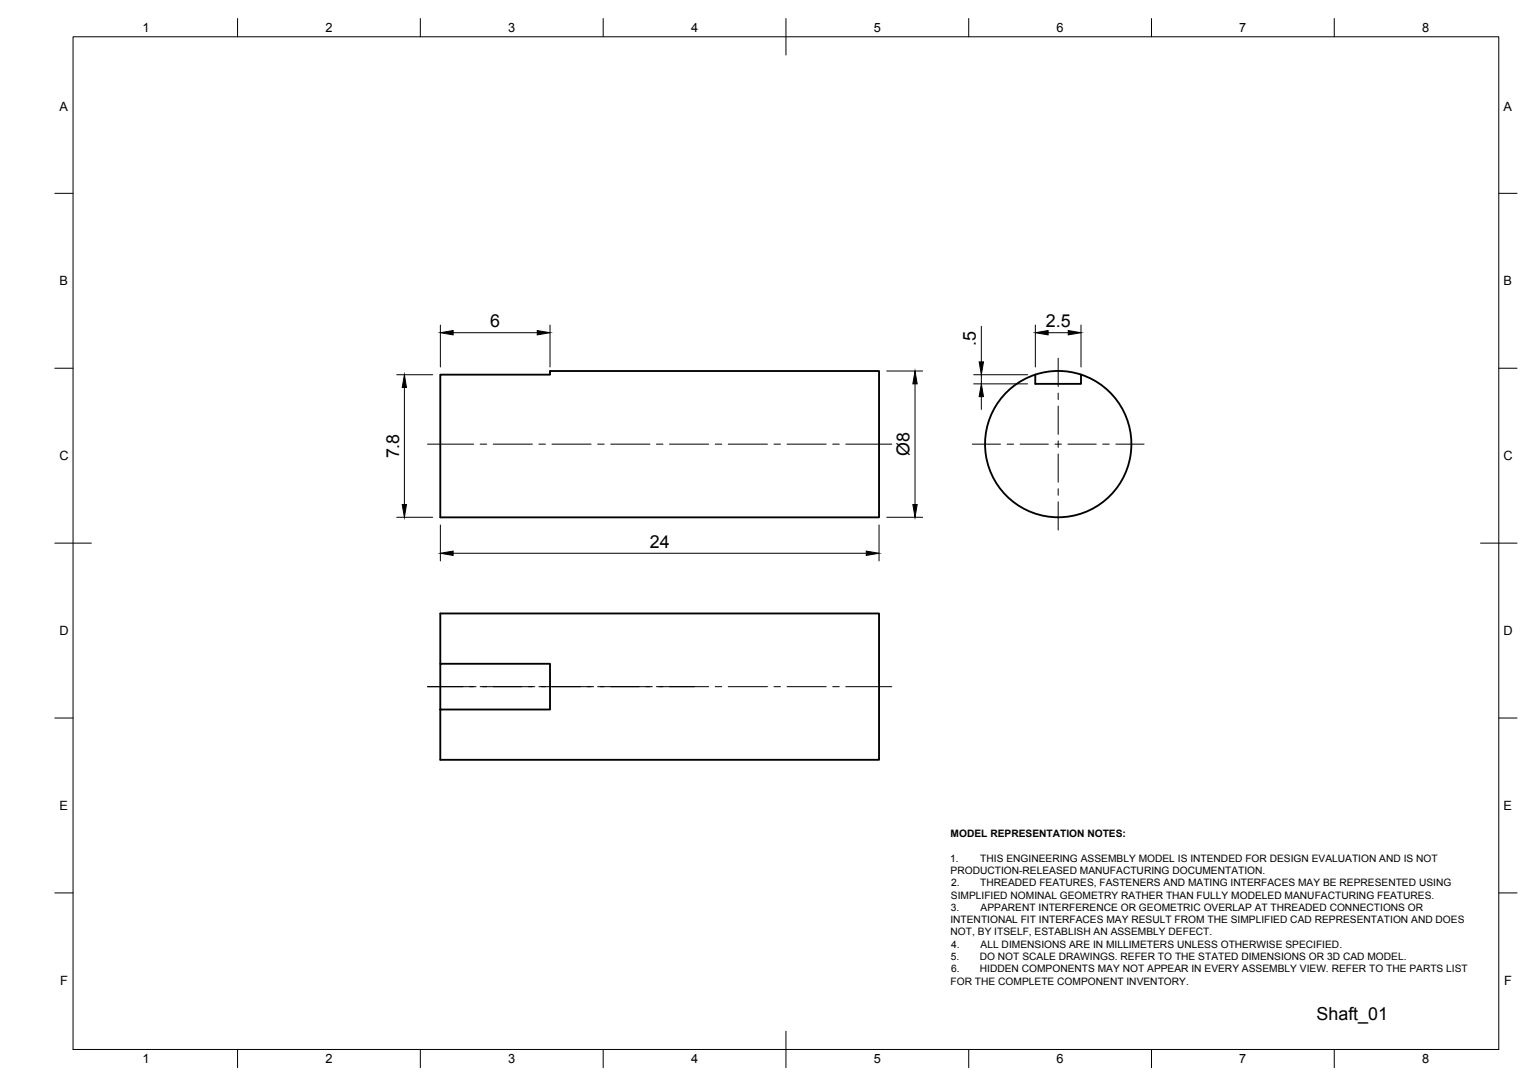
ISO-10303-21;
HEADER;
/* Generated by software containing ST-Developer
 * from STEP Tools, Inc. (www.steptools.com) 
 */

FILE_DESCRIPTION(
/* description */ (''),
/* implementation_level */ '2;1');

FILE_NAME(
/* name */ 'Shaft_01.step',
/* time_stamp */ '2026-10-05T22:24:12-07:00',
/* author */ (''),
/* organization */ (''),
/* preprocessor_version */ 'ST-DEVELOPER v20.2',
/* originating_system */ 'Autodesk Translation Framework v15.15.0.0',
/* authorisation */ '');

FILE_SCHEMA (('AUTOMOTIVE_DESIGN { 1 0 10303 214 3 1 1 }'));
ENDSEC;

DATA;
#10=MECHANICAL_DESIGN_GEOMETRIC_PRESENTATION_REPRESENTATION('',(#58),#2116);
#44=SHAPE_REPRESENTATION_RELATIONSHIP('SRR','None',#2150,#51);
#51=ADVANCED_BREP_SHAPE_REPRESENTATION('',(#65),#2114);
#58=STYLED_ITEM('',(#2192),#65);
#65=MANIFOLD_SOLID_BREP('Body1',#1152);
#119=PLANE('',#1329);
#120=PLANE('',#1330);
#121=PLANE('',#1332);
#122=PLANE('',#1333);
#123=PLANE('',#1338);
#124=PLANE('',#1339);
#185=FACE_OUTER_BOUND('',#260,.T.);
#186=FACE_OUTER_BOUND('',#261,.T.);
#187=FACE_OUTER_BOUND('',#262,.T.);
#188=FACE_OUTER_BOUND('',#263,.T.);
#189=FACE_OUTER_BOUND('',#264,.T.);
#190=FACE_OUTER_BOUND('',#265,.T.);
#191=FACE_OUTER_BOUND('',#266,.T.);
#260=EDGE_LOOP('',(#1015,#1016,#1017,#1018));
#261=EDGE_LOOP('',(#1019,#1020,#1021,#1022));
#262=EDGE_LOOP('',(#1023,#1024,#1025,#1026));
#263=EDGE_LOOP('',(#1027,#1028,#1029,#1030));
#264=EDGE_LOOP('',(#1031,#1032,#1033,#1034,#1035,#1036,#1037,#1038));
#265=EDGE_LOOP('',(#1039));
#266=EDGE_LOOP('',(#1040,#1041,#1042,#1043,#1044));
#358=LINE('',#2036,#463);
#359=LINE('',#2038,#464);
#360=LINE('',#2040,#465);
#361=LINE('',#2041,#466);
#362=LINE('',#2046,#467);
#363=LINE('',#2047,#468);
#364=LINE('',#2050,#469);
#365=LINE('',#2051,#470);
#366=LINE('',#2054,#471);
#367=LINE('',#2055,#472);
#368=LINE('',#2060,#473);
#463=VECTOR('',#1632,10.);
#464=VECTOR('',#1633,10.);
#465=VECTOR('',#1634,10.);
#466=VECTOR('',#1635,10.);
#467=VECTOR('',#1640,10.);
#468=VECTOR('',#1641,10.);
#469=VECTOR('',#1644,10.);
#470=VECTOR('',#1645,10.);
#471=VECTOR('',#1648,10.);
#472=VECTOR('',#1649,10.);
#473=VECTOR('',#1654,4.);
#522=CIRCLE('',#1331,4.);
#523=CIRCLE('',#1335,4.);
#524=CIRCLE('',#1336,4.);
#525=CIRCLE('',#1337,4.);
#607=VERTEX_POINT('',#2034);
#608=VERTEX_POINT('',#2035);
#609=VERTEX_POINT('',#2037);
#610=VERTEX_POINT('',#2039);
#611=VERTEX_POINT('',#2043);
#612=VERTEX_POINT('',#2045);
#613=VERTEX_POINT('',#2049);
#614=VERTEX_POINT('',#2053);
#615=VERTEX_POINT('',#2057);
#616=VERTEX_POINT('',#2059);
#746=EDGE_CURVE('',#607,#608,#358,.T.);
#747=EDGE_CURVE('',#609,#607,#359,.T.);
#748=EDGE_CURVE('',#609,#610,#360,.T.);
#749=EDGE_CURVE('',#610,#608,#361,.T.);
#750=EDGE_CURVE('',#608,#611,#522,.T.);
#751=EDGE_CURVE('',#612,#610,#362,.T.);
#752=EDGE_CURVE('',#611,#612,#363,.T.);
#753=EDGE_CURVE('',#613,#609,#364,.T.);
#754=EDGE_CURVE('',#613,#612,#365,.T.);
#755=EDGE_CURVE('',#611,#614,#366,.T.);
#756=EDGE_CURVE('',#614,#613,#367,.T.);
#757=EDGE_CURVE('',#615,#615,#523,.T.);
#758=EDGE_CURVE('',#615,#616,#368,.T.);
#759=EDGE_CURVE('',#616,#607,#524,.T.);
#760=EDGE_CURVE('',#614,#616,#525,.T.);
#1015=ORIENTED_EDGE('',*,*,#746,.F.);
#1016=ORIENTED_EDGE('',*,*,#747,.F.);
#1017=ORIENTED_EDGE('',*,*,#748,.T.);
#1018=ORIENTED_EDGE('',*,*,#749,.T.);
#1019=ORIENTED_EDGE('',*,*,#750,.F.);
#1020=ORIENTED_EDGE('',*,*,#749,.F.);
#1021=ORIENTED_EDGE('',*,*,#751,.F.);
#1022=ORIENTED_EDGE('',*,*,#752,.F.);
#1023=ORIENTED_EDGE('',*,*,#753,.F.);
#1024=ORIENTED_EDGE('',*,*,#754,.T.);
#1025=ORIENTED_EDGE('',*,*,#751,.T.);
#1026=ORIENTED_EDGE('',*,*,#748,.F.);
#1027=ORIENTED_EDGE('',*,*,#755,.F.);
#1028=ORIENTED_EDGE('',*,*,#752,.T.);
#1029=ORIENTED_EDGE('',*,*,#754,.F.);
#1030=ORIENTED_EDGE('',*,*,#756,.F.);
#1031=ORIENTED_EDGE('',*,*,#757,.F.);
#1032=ORIENTED_EDGE('',*,*,#758,.T.);
#1033=ORIENTED_EDGE('',*,*,#759,.T.);
#1034=ORIENTED_EDGE('',*,*,#746,.T.);
#1035=ORIENTED_EDGE('',*,*,#750,.T.);
#1036=ORIENTED_EDGE('',*,*,#755,.T.);
#1037=ORIENTED_EDGE('',*,*,#760,.T.);
#1038=ORIENTED_EDGE('',*,*,#758,.F.);
#1039=ORIENTED_EDGE('',*,*,#757,.T.);
#1040=ORIENTED_EDGE('',*,*,#747,.T.);
#1041=ORIENTED_EDGE('',*,*,#759,.F.);
#1042=ORIENTED_EDGE('',*,*,#760,.F.);
#1043=ORIENTED_EDGE('',*,*,#756,.T.);
#1044=ORIENTED_EDGE('',*,*,#753,.T.);
#1079=CYLINDRICAL_SURFACE('',#1334,4.);
#1134=ADVANCED_FACE('',(#185),#119,.F.);
#1135=ADVANCED_FACE('',(#186),#120,.F.);
#1136=ADVANCED_FACE('',(#187),#121,.F.);
#1137=ADVANCED_FACE('',(#188),#122,.F.);
#1138=ADVANCED_FACE('',(#189),#1079,.T.);
#1139=ADVANCED_FACE('',(#190),#123,.T.);
#1140=ADVANCED_FACE('',(#191),#124,.F.);
#1152=CLOSED_SHELL('',(#1134,#1135,#1136,#1137,#1138,#1139,#1140));
#1328=AXIS2_PLACEMENT_3D('',#2032,#1628,#1629);
#1329=AXIS2_PLACEMENT_3D('',#2033,#1630,#1631);
#1330=AXIS2_PLACEMENT_3D('',#2042,#1636,#1637);
#1331=AXIS2_PLACEMENT_3D('',#2044,#1638,#1639);
#1332=AXIS2_PLACEMENT_3D('',#2048,#1642,#1643);
#1333=AXIS2_PLACEMENT_3D('',#2052,#1646,#1647);
#1334=AXIS2_PLACEMENT_3D('',#2056,#1650,#1651);
#1335=AXIS2_PLACEMENT_3D('',#2058,#1652,#1653);
#1336=AXIS2_PLACEMENT_3D('',#2061,#1655,#1656);
#1337=AXIS2_PLACEMENT_3D('',#2062,#1657,#1658);
#1338=AXIS2_PLACEMENT_3D('',#2063,#1659,#1660);
#1339=AXIS2_PLACEMENT_3D('',#2064,#1661,#1662);
#1628=DIRECTION('axis',(0.,0.,1.));
#1629=DIRECTION('refdir',(1.,0.,0.));
#1630=DIRECTION('center_axis',(1.,0.,0.));
#1631=DIRECTION('ref_axis',(0.,0.,1.));
#1632=DIRECTION('',(0.,-1.,0.));
#1633=DIRECTION('',(0.,0.,1.));
#1634=DIRECTION('',(0.,-1.,0.));
#1635=DIRECTION('',(0.,0.,1.));
#1636=DIRECTION('center_axis',(0.,-1.,0.));
#1637=DIRECTION('ref_axis',(0.,0.,-1.));
#1638=DIRECTION('center_axis',(0.,-1.,0.));
#1639=DIRECTION('ref_axis',(1.,0.,0.));
#1640=DIRECTION('',(1.,0.,0.));
#1641=DIRECTION('',(0.,0.,-1.));
#1642=DIRECTION('center_axis',(0.,0.,-1.));
#1643=DIRECTION('ref_axis',(1.,0.,0.));
#1644=DIRECTION('',(1.,0.,0.));
#1645=DIRECTION('',(0.,-1.,0.));
#1646=DIRECTION('center_axis',(-1.,0.,0.));
#1647=DIRECTION('ref_axis',(0.,0.,-1.));
#1648=DIRECTION('',(0.,1.,0.));
#1649=DIRECTION('',(0.,0.,-1.));
#1650=DIRECTION('center_axis',(0.,-1.,0.));
#1651=DIRECTION('ref_axis',(1.,0.,0.));
#1652=DIRECTION('center_axis',(0.,-1.,0.));
#1653=DIRECTION('ref_axis',(1.,0.,0.));
#1654=DIRECTION('',(0.,1.,0.));
#1655=DIRECTION('center_axis',(0.,-1.,0.));
#1656=DIRECTION('ref_axis',(1.,0.,0.));
#1657=DIRECTION('center_axis',(0.,-1.,0.));
#1658=DIRECTION('ref_axis',(1.,0.,0.));
#1659=DIRECTION('center_axis',(0.,-1.,0.));
#1660=DIRECTION('ref_axis',(1.,0.,0.));
#1661=DIRECTION('center_axis',(0.,-1.,0.));
#1662=DIRECTION('ref_axis',(1.,0.,0.));
#2032=CARTESIAN_POINT('',(0.,0.,0.));
#2033=CARTESIAN_POINT('Origin',(1.25,-6.,3.29967103839267));
#2034=CARTESIAN_POINT('',(1.25,-6.,3.79967103839267));
#2035=CARTESIAN_POINT('',(1.25,-12.,3.79967103839267));
#2036=CARTESIAN_POINT('',(1.25,-6.,3.79967103839267));
#2037=CARTESIAN_POINT('',(1.25,-6.,3.29967103839267));
#2038=CARTESIAN_POINT('',(1.25,-6.,1.64983551919633));
#2039=CARTESIAN_POINT('',(1.25,-12.,3.29967103839267));
#2040=CARTESIAN_POINT('',(1.25,-6.,3.29967103839267));
#2041=CARTESIAN_POINT('',(1.25,-12.,6.32461990770089));
#2042=CARTESIAN_POINT('Origin',(0.,-12.,4.07045011057597));
#2043=CARTESIAN_POINT('',(-1.25,-12.,3.79967103839267));
#2044=CARTESIAN_POINT('Origin',(0.,-12.,0.));
#2045=CARTESIAN_POINT('',(-1.25,-12.,3.29967103839267));
#2046=CARTESIAN_POINT('',(-1.25,-12.,3.29967103839267));
#2047=CARTESIAN_POINT('',(-1.25,-12.,3.79967103839267));
#2048=CARTESIAN_POINT('Origin',(-1.25,-6.,3.29967103839267));
#2049=CARTESIAN_POINT('',(-1.25,-6.,3.29967103839267));
#2050=CARTESIAN_POINT('',(-0.625,-6.,3.29967103839267));
#2051=CARTESIAN_POINT('',(-1.25,-6.,3.29967103839267));
#2052=CARTESIAN_POINT('Origin',(-1.25,-6.,4.84122918275927));
#2053=CARTESIAN_POINT('',(-1.25,-6.,3.79967103839267));
#2054=CARTESIAN_POINT('',(-1.25,-6.,3.79967103839267));
#2055=CARTESIAN_POINT('',(-1.25,-6.,2.42061459137964));
#2056=CARTESIAN_POINT('Origin',(0.,-6.,0.));
#2057=CARTESIAN_POINT('',(-4.,-30.,-4.89858719658941E-16));
#2058=CARTESIAN_POINT('Origin',(0.,-30.,0.));
#2059=CARTESIAN_POINT('',(-4.,-6.,-4.89858719658941E-16));
#2060=CARTESIAN_POINT('',(-4.,-6.,-4.89858719658941E-16));
#2061=CARTESIAN_POINT('Origin',(0.,-6.,0.));
#2062=CARTESIAN_POINT('Origin',(0.,-6.,0.));
#2063=CARTESIAN_POINT('Origin',(0.,-30.,0.));
#2064=CARTESIAN_POINT('Origin',(0.,-6.,0.));
#2105=UNCERTAINTY_MEASURE_WITH_UNIT(LENGTH_MEASURE(0.01),#2117,
'DISTANCE_ACCURACY_VALUE',
'Maximum model space distance between geometric entities at asserted c
onnectivities');
#2107=UNCERTAINTY_MEASURE_WITH_UNIT(LENGTH_MEASURE(0.01),#2117,
'DISTANCE_ACCURACY_VALUE',
'Maximum model space distance between geometric entities at asserted c
onnectivities');
#2114=(
GEOMETRIC_REPRESENTATION_CONTEXT(3)
GLOBAL_UNCERTAINTY_ASSIGNED_CONTEXT((#2105))
GLOBAL_UNIT_ASSIGNED_CONTEXT((#2117,#2119,#2120))
REPRESENTATION_CONTEXT('','3D')
);
#2116=(
GEOMETRIC_REPRESENTATION_CONTEXT(3)
GLOBAL_UNCERTAINTY_ASSIGNED_CONTEXT((#2107))
GLOBAL_UNIT_ASSIGNED_CONTEXT((#2117,#2119,#2120))
REPRESENTATION_CONTEXT('','3D')
);
#2117=(
LENGTH_UNIT()
NAMED_UNIT(*)
SI_UNIT(.MILLI.,.METRE.)
);
#2119=(
NAMED_UNIT(*)
PLANE_ANGLE_UNIT()
SI_UNIT($,.RADIAN.)
);
#2120=(
NAMED_UNIT(*)
SI_UNIT($,.STERADIAN.)
SOLID_ANGLE_UNIT()
);
#2127=SHAPE_DEFINITION_REPRESENTATION(#2135,#2150);
#2135=PRODUCT_DEFINITION_SHAPE('',$,#2159);
#2150=SHAPE_REPRESENTATION('',(#1328),#2114);
#2152=PRODUCT_DEFINITION_CONTEXT('part definition',#2178,'design');
#2159=PRODUCT_DEFINITION('Shaft_01','Shaft_01',#2167,#2152);
#2167=PRODUCT_DEFINITION_FORMATION('',$,#2186);
#2178=APPLICATION_CONTEXT(
'Core Data for Automotive Mechanical Design Process');
#2179=PRODUCT_CONTEXT('part definition',#2178,'mechanical');
#2186=PRODUCT('Shaft_01','Shaft_01',$,(#2179));
#2192=PRESENTATION_STYLE_ASSIGNMENT((#2197));
#2197=SURFACE_STYLE_USAGE(.BOTH.,#2202);
#2202=SURFACE_SIDE_STYLE('',(#2207));
#2207=SURFACE_STYLE_FILL_AREA(#2212);
#2212=FILL_AREA_STYLE('Opaque(235,235,235)',(#2217));
#2217=FILL_AREA_STYLE_COLOUR('Opaque(235,235,235)',#2222);
#2222=COLOUR_RGB('Opaque(235,235,235)', 0.40784314, 0.44705882, 0.49803922);
ENDSEC;
END-ISO-10303-21;
